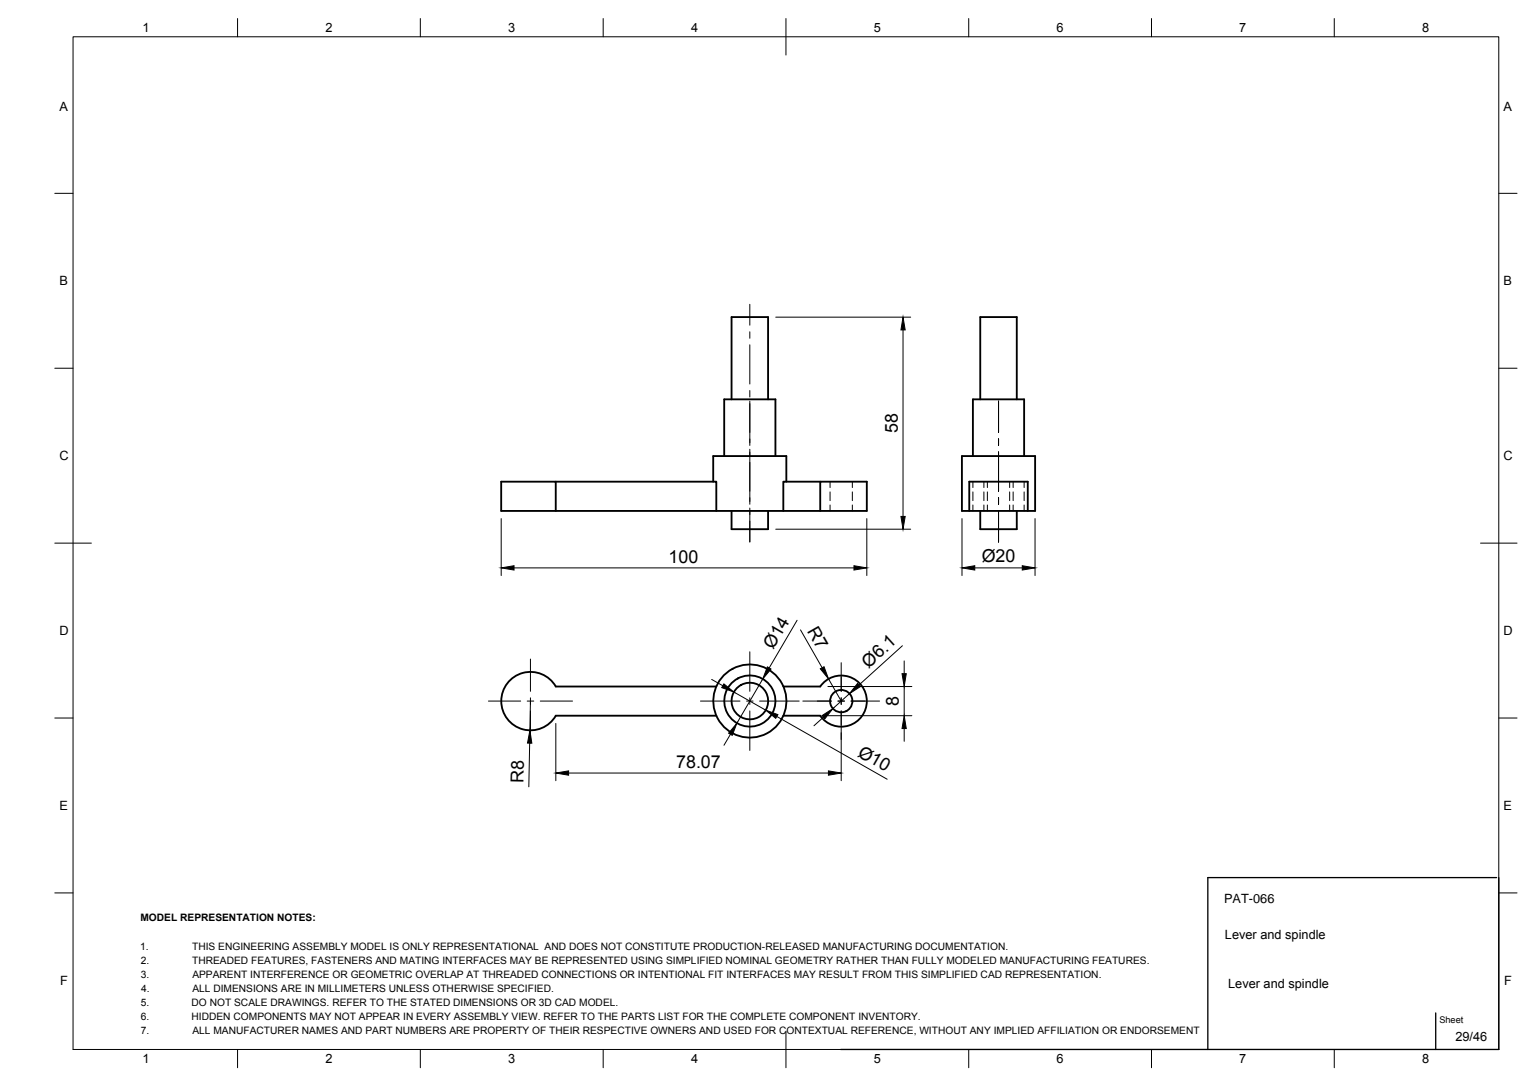
ISO-10303-21;
HEADER;
/* Generated by software containing ST-Developer
 * from STEP Tools, Inc. (www.steptools.com) 
 */

FILE_DESCRIPTION(
/* description */ ('Lever-operated bar clamp (toggle)'),
/* implementation_level */ '2;1');

FILE_NAME(
/* name */ 'Lever and spindle.step',
/* time_stamp */ '2026-10-28T03:25:02-07:00',
/* author */ (''),
/* organization */ (''),
/* preprocessor_version */ 'ST-DEVELOPER v20.2',
/* originating_system */ 'Autodesk Translation Framework v15.17.0.0',
/* authorisation */ '');

FILE_SCHEMA (('AUTOMOTIVE_DESIGN { 1 0 10303 214 3 1 1 }'));
ENDSEC;

DATA;
#10=MECHANICAL_DESIGN_GEOMETRIC_PRESENTATION_REPRESENTATION('',(#438),#12413);
#354=SHAPE_REPRESENTATION_RELATIONSHIP('SRR','None',#12596,#392);
#392=ADVANCED_BREP_SHAPE_REPRESENTATION('',(#483),#12393);
#438=STYLED_ITEM('',(#12862),#483);
#483=MANIFOLD_SOLID_BREP('Body1',#6599);
#610=FACE_BOUND('',#1653,.T.);
#611=FACE_BOUND('',#1654,.T.);
#612=FACE_BOUND('',#1661,.T.);
#613=FACE_BOUND('',#1664,.T.);
#614=FACE_BOUND('',#1667,.T.);
#785=PLANE('',#7551);
#786=PLANE('',#7557);
#787=PLANE('',#7558);
#788=PLANE('',#7560);
#789=PLANE('',#7563);
#790=PLANE('',#7564);
#791=PLANE('',#7566);
#792=PLANE('',#7567);
#793=PLANE('',#7571);
#794=PLANE('',#7579);
#795=PLANE('',#7580);
#1134=FACE_OUTER_BOUND('',#1650,.T.);
#1135=FACE_OUTER_BOUND('',#1651,.T.);
#1136=FACE_OUTER_BOUND('',#1652,.T.);
#1137=FACE_OUTER_BOUND('',#1655,.T.);
#1138=FACE_OUTER_BOUND('',#1656,.T.);
#1139=FACE_OUTER_BOUND('',#1657,.T.);
#1140=FACE_OUTER_BOUND('',#1658,.T.);
#1141=FACE_OUTER_BOUND('',#1659,.T.);
#1142=FACE_OUTER_BOUND('',#1660,.T.);
#1143=FACE_OUTER_BOUND('',#1662,.T.);
#1144=FACE_OUTER_BOUND('',#1663,.T.);
#1145=FACE_OUTER_BOUND('',#1665,.T.);
#1146=FACE_OUTER_BOUND('',#1666,.T.);
#1147=FACE_OUTER_BOUND('',#1668,.T.);
#1148=FACE_OUTER_BOUND('',#1669,.T.);
#1149=FACE_OUTER_BOUND('',#1670,.T.);
#1150=FACE_OUTER_BOUND('',#1671,.T.);
#1151=FACE_OUTER_BOUND('',#1672,.T.);
#1650=EDGE_LOOP('',(#5423,#5424,#5425,#5426));
#1651=EDGE_LOOP('',(#5427,#5428,#5429,#5430));
#1652=EDGE_LOOP('',(#5431,#5432,#5433,#5434,#5435,#5436,#5437,#5438,#5439));
#1653=EDGE_LOOP('',(#5440));
#1654=EDGE_LOOP('',(#5441));
#1655=EDGE_LOOP('',(#5442,#5443,#5444,#5445));
#1656=EDGE_LOOP('',(#5446,#5447,#5448,#5449));
#1657=EDGE_LOOP('',(#5450,#5451,#5452,#5453));
#1658=EDGE_LOOP('',(#5454,#5455,#5456,#5457));
#1659=EDGE_LOOP('',(#5458,#5459,#5460,#5461));
#1660=EDGE_LOOP('',(#5462,#5463,#5464,#5465));
#1661=EDGE_LOOP('',(#5466));
#1662=EDGE_LOOP('',(#5467,#5468,#5469,#5470));
#1663=EDGE_LOOP('',(#5471));
#1664=EDGE_LOOP('',(#5472));
#1665=EDGE_LOOP('',(#5473,#5474,#5475,#5476,#5477,#5478,#5479,#5480,#5481,
#5482,#5483,#5484));
#1666=EDGE_LOOP('',(#5485));
#1667=EDGE_LOOP('',(#5486));
#1668=EDGE_LOOP('',(#5487,#5488,#5489,#5490));
#1669=EDGE_LOOP('',(#5491,#5492,#5493,#5494));
#1670=EDGE_LOOP('',(#5495,#5496,#5497,#5498));
#1671=EDGE_LOOP('',(#5499));
#1672=EDGE_LOOP('',(#5500));
#2107=LINE('',#11508,#2548);
#2108=LINE('',#11513,#2549);
#2109=LINE('',#11517,#2550);
#2110=LINE('',#11521,#2551);
#2111=LINE('',#11527,#2552);
#2112=LINE('',#11531,#2553);
#2113=LINE('',#11534,#2554);
#2114=LINE('',#11539,#2555);
#2115=LINE('',#11540,#2556);
#2116=LINE('',#11543,#2557);
#2117=LINE('',#11546,#2558);
#2118=LINE('',#11549,#2559);
#2119=LINE('',#11552,#2560);
#2120=LINE('',#11555,#2561);
#2121=LINE('',#11556,#2562);
#2122=LINE('',#11559,#2563);
#2123=LINE('',#11562,#2564);
#2124=LINE('',#11569,#2565);
#2125=LINE('',#11576,#2566);
#2126=LINE('',#11579,#2567);
#2127=LINE('',#11584,#2568);
#2548=VECTOR('',#9166,0.305);
#2549=VECTOR('',#9171,1.);
#2550=VECTOR('',#9174,1.);
#2551=VECTOR('',#9179,1.);
#2552=VECTOR('',#9184,1.);
#2553=VECTOR('',#9187,1.);
#2554=VECTOR('',#9190,1.);
#2555=VECTOR('',#9195,1.);
#2556=VECTOR('',#9196,1.);
#2557=VECTOR('',#9199,1.);
#2558=VECTOR('',#9204,1.);
#2559=VECTOR('',#9207,1.);
#2560=VECTOR('',#9210,1.);
#2561=VECTOR('',#9213,1.);
#2562=VECTOR('',#9214,1.);
#2563=VECTOR('',#9217,1.);
#2564=VECTOR('',#9222,1.);
#2565=VECTOR('',#9231,1.);
#2566=VECTOR('',#9240,0.7);
#2567=VECTOR('',#9243,0.5);
#2568=VECTOR('',#9250,0.5);
#2960=CIRCLE('',#7546,0.305);
#2961=CIRCLE('',#7547,0.305);
#2962=CIRCLE('',#7549,0.8);
#2963=CIRCLE('',#7550,0.8);
#2964=CIRCLE('',#7552,1.);
#2965=CIRCLE('',#7553,1.);
#2966=CIRCLE('',#7554,0.7);
#2967=CIRCLE('',#7555,1.);
#2968=CIRCLE('',#7556,0.5);
#2969=CIRCLE('',#7559,1.);
#2970=CIRCLE('',#7562,0.7);
#2971=CIRCLE('',#7565,1.);
#2972=CIRCLE('',#7568,1.);
#2973=CIRCLE('',#7569,0.7);
#2974=CIRCLE('',#7572,0.7);
#2975=CIRCLE('',#7573,0.5);
#2976=CIRCLE('',#7576,0.5);
#2977=CIRCLE('',#7578,0.5);
#3415=VERTEX_POINT('',#11505);
#3416=VERTEX_POINT('',#11507);
#3417=VERTEX_POINT('',#11511);
#3418=VERTEX_POINT('',#11512);
#3419=VERTEX_POINT('',#11514);
#3420=VERTEX_POINT('',#11516);
#3421=VERTEX_POINT('',#11520);
#3422=VERTEX_POINT('',#11522);
#3423=VERTEX_POINT('',#11524);
#3424=VERTEX_POINT('',#11526);
#3425=VERTEX_POINT('',#11528);
#3426=VERTEX_POINT('',#11530);
#3427=VERTEX_POINT('',#11532);
#3428=VERTEX_POINT('',#11535);
#3429=VERTEX_POINT('',#11538);
#3430=VERTEX_POINT('',#11542);
#3431=VERTEX_POINT('',#11548);
#3432=VERTEX_POINT('',#11550);
#3433=VERTEX_POINT('',#11554);
#3434=VERTEX_POINT('',#11558);
#3435=VERTEX_POINT('',#11564);
#3436=VERTEX_POINT('',#11566);
#3437=VERTEX_POINT('',#11571);
#3438=VERTEX_POINT('',#11573);
#3439=VERTEX_POINT('',#11578);
#3440=VERTEX_POINT('',#11582);
#4116=EDGE_CURVE('',#3415,#3415,#2960,.T.);
#4117=EDGE_CURVE('',#3415,#3416,#2107,.T.);
#4118=EDGE_CURVE('',#3416,#3416,#2961,.T.);
#4119=EDGE_CURVE('',#3417,#3418,#2108,.T.);
#4120=EDGE_CURVE('',#3419,#3417,#2962,.T.);
#4121=EDGE_CURVE('',#3420,#3419,#2109,.T.);
#4122=EDGE_CURVE('',#3420,#3418,#2963,.T.);
#4123=EDGE_CURVE('',#3421,#3420,#2110,.T.);
#4124=EDGE_CURVE('',#3422,#3421,#2964,.T.);
#4125=EDGE_CURVE('',#3423,#3422,#2965,.T.);
#4126=EDGE_CURVE('',#3424,#3423,#2111,.T.);
#4127=EDGE_CURVE('',#3425,#3424,#2966,.T.);
#4128=EDGE_CURVE('',#3426,#3425,#2112,.T.);
#4129=EDGE_CURVE('',#3427,#3426,#2967,.T.);
#4130=EDGE_CURVE('',#3418,#3427,#2113,.T.);
#4131=EDGE_CURVE('',#3428,#3428,#2968,.T.);
#4132=EDGE_CURVE('',#3429,#3419,#2114,.T.);
#4133=EDGE_CURVE('',#3421,#3429,#2115,.T.);
#4134=EDGE_CURVE('',#3417,#3430,#2116,.T.);
#4135=EDGE_CURVE('',#3429,#3430,#2969,.T.);
#4136=EDGE_CURVE('',#3430,#3427,#2117,.T.);
#4137=EDGE_CURVE('',#3431,#3424,#2118,.T.);
#4138=EDGE_CURVE('',#3432,#3431,#2970,.T.);
#4139=EDGE_CURVE('',#3425,#3432,#2119,.T.);
#4140=EDGE_CURVE('',#3433,#3432,#2120,.T.);
#4141=EDGE_CURVE('',#3426,#3433,#2121,.T.);
#4142=EDGE_CURVE('',#3431,#3434,#2122,.T.);
#4143=EDGE_CURVE('',#3433,#3434,#2971,.T.);
#4144=EDGE_CURVE('',#3434,#3423,#2123,.T.);
#4145=EDGE_CURVE('',#3435,#3435,#2972,.T.);
#4146=EDGE_CURVE('',#3436,#3436,#2973,.T.);
#4147=EDGE_CURVE('',#3435,#3422,#2124,.T.);
#4148=EDGE_CURVE('',#3437,#3437,#2974,.T.);
#4149=EDGE_CURVE('',#3438,#3438,#2975,.T.);
#4150=EDGE_CURVE('',#3437,#3436,#2125,.T.);
#4151=EDGE_CURVE('',#3428,#3439,#2126,.T.);
#4152=EDGE_CURVE('',#3439,#3439,#2976,.T.);
#4153=EDGE_CURVE('',#3440,#3440,#2977,.T.);
#4154=EDGE_CURVE('',#3440,#3438,#2127,.T.);
#5423=ORIENTED_EDGE('',*,*,#4116,.F.);
#5424=ORIENTED_EDGE('',*,*,#4117,.T.);
#5425=ORIENTED_EDGE('',*,*,#4118,.F.);
#5426=ORIENTED_EDGE('',*,*,#4117,.F.);
#5427=ORIENTED_EDGE('',*,*,#4119,.F.);
#5428=ORIENTED_EDGE('',*,*,#4120,.F.);
#5429=ORIENTED_EDGE('',*,*,#4121,.F.);
#5430=ORIENTED_EDGE('',*,*,#4122,.T.);
#5431=ORIENTED_EDGE('',*,*,#4122,.F.);
#5432=ORIENTED_EDGE('',*,*,#4123,.F.);
#5433=ORIENTED_EDGE('',*,*,#4124,.F.);
#5434=ORIENTED_EDGE('',*,*,#4125,.F.);
#5435=ORIENTED_EDGE('',*,*,#4126,.F.);
#5436=ORIENTED_EDGE('',*,*,#4127,.F.);
#5437=ORIENTED_EDGE('',*,*,#4128,.F.);
#5438=ORIENTED_EDGE('',*,*,#4129,.F.);
#5439=ORIENTED_EDGE('',*,*,#4130,.F.);
#5440=ORIENTED_EDGE('',*,*,#4116,.T.);
#5441=ORIENTED_EDGE('',*,*,#4131,.F.);
#5442=ORIENTED_EDGE('',*,*,#4121,.T.);
#5443=ORIENTED_EDGE('',*,*,#4132,.F.);
#5444=ORIENTED_EDGE('',*,*,#4133,.F.);
#5445=ORIENTED_EDGE('',*,*,#4123,.T.);
#5446=ORIENTED_EDGE('',*,*,#4134,.T.);
#5447=ORIENTED_EDGE('',*,*,#4135,.F.);
#5448=ORIENTED_EDGE('',*,*,#4132,.T.);
#5449=ORIENTED_EDGE('',*,*,#4120,.T.);
#5450=ORIENTED_EDGE('',*,*,#4119,.T.);
#5451=ORIENTED_EDGE('',*,*,#4130,.T.);
#5452=ORIENTED_EDGE('',*,*,#4136,.F.);
#5453=ORIENTED_EDGE('',*,*,#4134,.F.);
#5454=ORIENTED_EDGE('',*,*,#4137,.F.);
#5455=ORIENTED_EDGE('',*,*,#4138,.F.);
#5456=ORIENTED_EDGE('',*,*,#4139,.F.);
#5457=ORIENTED_EDGE('',*,*,#4127,.T.);
#5458=ORIENTED_EDGE('',*,*,#4139,.T.);
#5459=ORIENTED_EDGE('',*,*,#4140,.F.);
#5460=ORIENTED_EDGE('',*,*,#4141,.F.);
#5461=ORIENTED_EDGE('',*,*,#4128,.T.);
#5462=ORIENTED_EDGE('',*,*,#4142,.T.);
#5463=ORIENTED_EDGE('',*,*,#4143,.F.);
#5464=ORIENTED_EDGE('',*,*,#4140,.T.);
#5465=ORIENTED_EDGE('',*,*,#4138,.T.);
#5466=ORIENTED_EDGE('',*,*,#4118,.T.);
#5467=ORIENTED_EDGE('',*,*,#4137,.T.);
#5468=ORIENTED_EDGE('',*,*,#4126,.T.);
#5469=ORIENTED_EDGE('',*,*,#4144,.F.);
#5470=ORIENTED_EDGE('',*,*,#4142,.F.);
#5471=ORIENTED_EDGE('',*,*,#4145,.T.);
#5472=ORIENTED_EDGE('',*,*,#4146,.F.);
#5473=ORIENTED_EDGE('',*,*,#4145,.F.);
#5474=ORIENTED_EDGE('',*,*,#4147,.T.);
#5475=ORIENTED_EDGE('',*,*,#4124,.T.);
#5476=ORIENTED_EDGE('',*,*,#4133,.T.);
#5477=ORIENTED_EDGE('',*,*,#4135,.T.);
#5478=ORIENTED_EDGE('',*,*,#4136,.T.);
#5479=ORIENTED_EDGE('',*,*,#4129,.T.);
#5480=ORIENTED_EDGE('',*,*,#4141,.T.);
#5481=ORIENTED_EDGE('',*,*,#4143,.T.);
#5482=ORIENTED_EDGE('',*,*,#4144,.T.);
#5483=ORIENTED_EDGE('',*,*,#4125,.T.);
#5484=ORIENTED_EDGE('',*,*,#4147,.F.);
#5485=ORIENTED_EDGE('',*,*,#4148,.T.);
#5486=ORIENTED_EDGE('',*,*,#4149,.F.);
#5487=ORIENTED_EDGE('',*,*,#4148,.F.);
#5488=ORIENTED_EDGE('',*,*,#4150,.T.);
#5489=ORIENTED_EDGE('',*,*,#4146,.T.);
#5490=ORIENTED_EDGE('',*,*,#4150,.F.);
#5491=ORIENTED_EDGE('',*,*,#4131,.T.);
#5492=ORIENTED_EDGE('',*,*,#4151,.T.);
#5493=ORIENTED_EDGE('',*,*,#4152,.T.);
#5494=ORIENTED_EDGE('',*,*,#4151,.F.);
#5495=ORIENTED_EDGE('',*,*,#4153,.F.);
#5496=ORIENTED_EDGE('',*,*,#4154,.T.);
#5497=ORIENTED_EDGE('',*,*,#4149,.T.);
#5498=ORIENTED_EDGE('',*,*,#4154,.F.);
#5499=ORIENTED_EDGE('',*,*,#4153,.T.);
#5500=ORIENTED_EDGE('',*,*,#4152,.F.);
#6116=CYLINDRICAL_SURFACE('',#7545,0.305);
#6117=CYLINDRICAL_SURFACE('',#7548,0.8);
#6118=CYLINDRICAL_SURFACE('',#7561,0.7);
#6119=CYLINDRICAL_SURFACE('',#7570,1.);
#6120=CYLINDRICAL_SURFACE('',#7574,0.7);
#6121=CYLINDRICAL_SURFACE('',#7575,0.5);
#6122=CYLINDRICAL_SURFACE('',#7577,0.5);
#6409=ADVANCED_FACE('',(#1134),#6116,.F.);
#6410=ADVANCED_FACE('',(#1135),#6117,.T.);
#6411=ADVANCED_FACE('',(#1136,#610,#611),#785,.F.);
#6412=ADVANCED_FACE('',(#1137),#786,.T.);
#6413=ADVANCED_FACE('',(#1138),#787,.T.);
#6414=ADVANCED_FACE('',(#1139),#788,.T.);
#6415=ADVANCED_FACE('',(#1140),#6118,.T.);
#6416=ADVANCED_FACE('',(#1141),#789,.T.);
#6417=ADVANCED_FACE('',(#1142,#612),#790,.T.);
#6418=ADVANCED_FACE('',(#1143),#791,.T.);
#6419=ADVANCED_FACE('',(#1144,#613),#792,.T.);
#6420=ADVANCED_FACE('',(#1145),#6119,.T.);
#6421=ADVANCED_FACE('',(#1146,#614),#793,.T.);
#6422=ADVANCED_FACE('',(#1147),#6120,.T.);
#6423=ADVANCED_FACE('',(#1148),#6121,.T.);
#6424=ADVANCED_FACE('',(#1149),#6122,.T.);
#6425=ADVANCED_FACE('',(#1150),#794,.T.);
#6426=ADVANCED_FACE('',(#1151),#795,.F.);
#6599=CLOSED_SHELL('',(#6409,#6410,#6411,#6412,#6413,#6414,#6415,#6416,
#6417,#6418,#6419,#6420,#6421,#6422,#6423,#6424,#6425,#6426));
#7544=AXIS2_PLACEMENT_3D('',#11503,#9160,#9161);
#7545=AXIS2_PLACEMENT_3D('',#11504,#9162,#9163);
#7546=AXIS2_PLACEMENT_3D('',#11506,#9164,#9165);
#7547=AXIS2_PLACEMENT_3D('',#11509,#9167,#9168);
#7548=AXIS2_PLACEMENT_3D('',#11510,#9169,#9170);
#7549=AXIS2_PLACEMENT_3D('',#11515,#9172,#9173);
#7550=AXIS2_PLACEMENT_3D('',#11518,#9175,#9176);
#7551=AXIS2_PLACEMENT_3D('',#11519,#9177,#9178);
#7552=AXIS2_PLACEMENT_3D('',#11523,#9180,#9181);
#7553=AXIS2_PLACEMENT_3D('',#11525,#9182,#9183);
#7554=AXIS2_PLACEMENT_3D('',#11529,#9185,#9186);
#7555=AXIS2_PLACEMENT_3D('',#11533,#9188,#9189);
#7556=AXIS2_PLACEMENT_3D('',#11536,#9191,#9192);
#7557=AXIS2_PLACEMENT_3D('',#11537,#9193,#9194);
#7558=AXIS2_PLACEMENT_3D('',#11541,#9197,#9198);
#7559=AXIS2_PLACEMENT_3D('',#11544,#9200,#9201);
#7560=AXIS2_PLACEMENT_3D('',#11545,#9202,#9203);
#7561=AXIS2_PLACEMENT_3D('',#11547,#9205,#9206);
#7562=AXIS2_PLACEMENT_3D('',#11551,#9208,#9209);
#7563=AXIS2_PLACEMENT_3D('',#11553,#9211,#9212);
#7564=AXIS2_PLACEMENT_3D('',#11557,#9215,#9216);
#7565=AXIS2_PLACEMENT_3D('',#11560,#9218,#9219);
#7566=AXIS2_PLACEMENT_3D('',#11561,#9220,#9221);
#7567=AXIS2_PLACEMENT_3D('',#11563,#9223,#9224);
#7568=AXIS2_PLACEMENT_3D('',#11565,#9225,#9226);
#7569=AXIS2_PLACEMENT_3D('',#11567,#9227,#9228);
#7570=AXIS2_PLACEMENT_3D('',#11568,#9229,#9230);
#7571=AXIS2_PLACEMENT_3D('',#11570,#9232,#9233);
#7572=AXIS2_PLACEMENT_3D('',#11572,#9234,#9235);
#7573=AXIS2_PLACEMENT_3D('',#11574,#9236,#9237);
#7574=AXIS2_PLACEMENT_3D('',#11575,#9238,#9239);
#7575=AXIS2_PLACEMENT_3D('',#11577,#9241,#9242);
#7576=AXIS2_PLACEMENT_3D('',#11580,#9244,#9245);
#7577=AXIS2_PLACEMENT_3D('',#11581,#9246,#9247);
#7578=AXIS2_PLACEMENT_3D('',#11583,#9248,#9249);
#7579=AXIS2_PLACEMENT_3D('',#11585,#9251,#9252);
#7580=AXIS2_PLACEMENT_3D('',#11586,#9253,#9254);
#9160=DIRECTION('axis',(0.,0.,1.));
#9161=DIRECTION('refdir',(1.,0.,0.));
#9162=DIRECTION('center_axis',(0.,1.,0.));
#9163=DIRECTION('ref_axis',(1.,0.,0.));
#9164=DIRECTION('center_axis',(0.,1.,0.));
#9165=DIRECTION('ref_axis',(1.,0.,0.));
#9166=DIRECTION('',(0.,1.,0.));
#9167=DIRECTION('center_axis',(0.,-1.,0.));
#9168=DIRECTION('ref_axis',(1.,0.,0.));
#9169=DIRECTION('center_axis',(0.,1.,0.));
#9170=DIRECTION('ref_axis',(-0.46947156278589,0.,0.882947592858928));
#9171=DIRECTION('',(0.,-1.,0.));
#9172=DIRECTION('center_axis',(0.,1.,0.));
#9173=DIRECTION('ref_axis',(1.,0.,0.));
#9174=DIRECTION('',(0.,1.,0.));
#9175=DIRECTION('center_axis',(0.,1.,0.));
#9176=DIRECTION('ref_axis',(1.,0.,0.));
#9177=DIRECTION('center_axis',(0.,1.,0.));
#9178=DIRECTION('ref_axis',(1.,0.,0.));
#9179=DIRECTION('',(-0.469471562785891,0.,0.882947592858927));
#9180=DIRECTION('center_axis',(0.,1.,0.));
#9181=DIRECTION('ref_axis',(1.,0.,0.));
#9182=DIRECTION('center_axis',(0.,1.,0.));
#9183=DIRECTION('ref_axis',(1.,0.,0.));
#9184=DIRECTION('',(-0.469471562785891,0.,0.882947592858927));
#9185=DIRECTION('center_axis',(0.,1.,0.));
#9186=DIRECTION('ref_axis',(1.,0.,0.));
#9187=DIRECTION('',(0.469471562785891,0.,-0.882947592858927));
#9188=DIRECTION('center_axis',(0.,1.,0.));
#9189=DIRECTION('ref_axis',(1.,0.,0.));
#9190=DIRECTION('',(0.469471562785891,0.,-0.882947592858927));
#9191=DIRECTION('center_axis',(0.,-1.,0.));
#9192=DIRECTION('ref_axis',(1.,0.,0.));
#9193=DIRECTION('center_axis',(-0.882947592858927,0.,-0.469471562785891));
#9194=DIRECTION('ref_axis',(-0.469471562785891,0.,0.882947592858927));
#9195=DIRECTION('',(-0.469471562785891,0.,0.882947592858927));
#9196=DIRECTION('',(0.,1.,0.));
#9197=DIRECTION('center_axis',(0.,1.,0.));
#9198=DIRECTION('ref_axis',(0.,0.,1.));
#9199=DIRECTION('',(0.469471562785891,0.,-0.882947592858927));
#9200=DIRECTION('center_axis',(0.,1.,0.));
#9201=DIRECTION('ref_axis',(1.,0.,0.));
#9202=DIRECTION('center_axis',(0.882947592858927,0.,0.469471562785891));
#9203=DIRECTION('ref_axis',(0.469471562785891,0.,-0.882947592858927));
#9204=DIRECTION('',(0.,-1.,0.));
#9205=DIRECTION('center_axis',(0.,1.,0.));
#9206=DIRECTION('ref_axis',(0.46947156278589,0.,-0.882947592858927));
#9207=DIRECTION('',(0.,-1.,0.));
#9208=DIRECTION('center_axis',(0.,1.,0.));
#9209=DIRECTION('ref_axis',(1.,0.,0.));
#9210=DIRECTION('',(0.,1.,0.));
#9211=DIRECTION('center_axis',(0.882947592858927,0.,0.469471562785891));
#9212=DIRECTION('ref_axis',(0.469471562785891,0.,-0.882947592858927));
#9213=DIRECTION('',(0.469471562785891,0.,-0.882947592858927));
#9214=DIRECTION('',(0.,1.,0.));
#9215=DIRECTION('center_axis',(0.,1.,0.));
#9216=DIRECTION('ref_axis',(0.,0.,1.));
#9217=DIRECTION('',(-0.469471562785891,0.,0.882947592858927));
#9218=DIRECTION('center_axis',(0.,1.,0.));
#9219=DIRECTION('ref_axis',(1.,0.,0.));
#9220=DIRECTION('center_axis',(-0.882947592858927,0.,-0.469471562785891));
#9221=DIRECTION('ref_axis',(-0.469471562785891,0.,0.882947592858927));
#9222=DIRECTION('',(0.,-1.,0.));
#9223=DIRECTION('center_axis',(0.,1.,0.));
#9224=DIRECTION('ref_axis',(1.,0.,0.));
#9225=DIRECTION('center_axis',(0.,1.,0.));
#9226=DIRECTION('ref_axis',(1.,0.,0.));
#9227=DIRECTION('center_axis',(0.,1.,0.));
#9228=DIRECTION('ref_axis',(1.,0.,0.));
#9229=DIRECTION('center_axis',(0.,1.,0.));
#9230=DIRECTION('ref_axis',(1.,0.,0.));
#9231=DIRECTION('',(0.,-1.,0.));
#9232=DIRECTION('center_axis',(0.,1.,0.));
#9233=DIRECTION('ref_axis',(1.,0.,0.));
#9234=DIRECTION('center_axis',(0.,1.,0.));
#9235=DIRECTION('ref_axis',(1.,0.,0.));
#9236=DIRECTION('center_axis',(0.,1.,0.));
#9237=DIRECTION('ref_axis',(1.,0.,0.));
#9238=DIRECTION('center_axis',(0.,1.,0.));
#9239=DIRECTION('ref_axis',(1.,0.,0.));
#9240=DIRECTION('',(0.,-1.,0.));
#9241=DIRECTION('center_axis',(0.,1.,0.));
#9242=DIRECTION('ref_axis',(1.,0.,0.));
#9243=DIRECTION('',(0.,-1.,0.));
#9244=DIRECTION('center_axis',(0.,1.,0.));
#9245=DIRECTION('ref_axis',(1.,0.,0.));
#9246=DIRECTION('center_axis',(0.,1.,0.));
#9247=DIRECTION('ref_axis',(1.,0.,0.));
#9248=DIRECTION('center_axis',(0.,1.,0.));
#9249=DIRECTION('ref_axis',(1.,0.,0.));
#9250=DIRECTION('',(0.,-1.,0.));
#9251=DIRECTION('center_axis',(0.,1.,0.));
#9252=DIRECTION('ref_axis',(1.,0.,0.));
#9253=DIRECTION('center_axis',(0.,1.,0.));
#9254=DIRECTION('ref_axis',(1.,0.,0.));
#11503=CARTESIAN_POINT('',(0.,0.,0.));
#11504=CARTESIAN_POINT('Origin',(-2.82632109303527,-3.6,8.79263101785268));
#11505=CARTESIAN_POINT('',(-3.13132109303527,-3.5,8.79263101785268));
#11506=CARTESIAN_POINT('Origin',(-2.82632109303527,-3.5,8.79263101785268));
#11507=CARTESIAN_POINT('',(-3.13132109303527,-2.7,8.79263101785268));
#11508=CARTESIAN_POINT('',(-3.13132109303527,-3.6,8.79263101785268));
#11509=CARTESIAN_POINT('Origin',(-2.82632109303527,-2.7,8.79263101785268));
#11510=CARTESIAN_POINT('Origin',(-6.81682937671534,-3.5,16.2976855571536));
#11511=CARTESIAN_POINT('',(-6.1383908997902,-2.7,15.873750145767));
#11512=CARTESIAN_POINT('',(-6.1383908997902,-3.5,15.873750145767));
#11513=CARTESIAN_POINT('',(-6.1383908997902,-3.5,15.873750145767));
#11514=CARTESIAN_POINT('',(-6.84474897407734,-2.7,15.4981728955383));
#11515=CARTESIAN_POINT('Origin',(-6.81682937671534,-2.7,16.2976855571536));
#11516=CARTESIAN_POINT('',(-6.84474897407734,-3.5,15.4981728955383));
#11517=CARTESIAN_POINT('',(-6.84474897407734,-3.5,15.4981728955383));
#11518=CARTESIAN_POINT('Origin',(-6.81682937671534,-3.5,16.2976855571536));
#11519=CARTESIAN_POINT('Origin',(-4.,-3.5,11.));
#11520=CARTESIAN_POINT('',(-4.78345683176268,-3.5,11.6214462106767));
#11521=CARTESIAN_POINT('',(-4.35317903714357,-3.5,10.8122113748856));
#11522=CARTESIAN_POINT('',(-5.,-3.5,11.));
#11523=CARTESIAN_POINT('Origin',(-4.,-3.5,11.));
#11524=CARTESIAN_POINT('',(-3.92290124252446,-3.5,10.0029765390946));
#11525=CARTESIAN_POINT('Origin',(-4.,-3.5,11.));
#11526=CARTESIAN_POINT('',(-3.44919101049801,-3.5,9.11205716881713));
#11527=CARTESIAN_POINT('',(-3.17950013017884,-3.5,8.60484239273833));
#11528=CARTESIAN_POINT('',(-2.74283293621087,-3.5,9.48763441904585));
#11529=CARTESIAN_POINT('Origin',(-2.82632109303527,-3.5,8.79263101785268));
#11530=CARTESIAN_POINT('',(-3.21654316823732,-3.5,10.3785537893233));
#11531=CARTESIAN_POINT('',(-3.64682096285643,-3.5,11.1877886251144));
#11532=CARTESIAN_POINT('',(-4.07709875747554,-3.5,11.9970234609054));
#11533=CARTESIAN_POINT('Origin',(-4.,-3.5,11.));
#11534=CARTESIAN_POINT('',(-6.46365033957177,-3.5,16.4854741822679));
#11535=CARTESIAN_POINT('',(-4.5,-3.5,11.));
#11536=CARTESIAN_POINT('Origin',(-4.,-3.5,11.));
#11537=CARTESIAN_POINT('Origin',(-4.35317903714357,-3.5,10.8122113748856));
#11538=CARTESIAN_POINT('',(-4.78345683176268,-2.7,11.6214462106767));
#11539=CARTESIAN_POINT('',(-4.35317903714357,-2.7,10.8122113748856));
#11540=CARTESIAN_POINT('',(-4.78345683176268,-3.5,11.6214462106767));
#11541=CARTESIAN_POINT('Origin',(-5.40841468835767,-2.7,13.6488427785768));
#11542=CARTESIAN_POINT('',(-4.07709875747554,-2.7,11.9970234609054));
#11543=CARTESIAN_POINT('',(-6.46365033957177,-2.7,16.4854741822679));
#11544=CARTESIAN_POINT('Origin',(-4.,-2.7,11.));
#11545=CARTESIAN_POINT('Origin',(-6.46365033957177,-3.5,16.4854741822679));
#11546=CARTESIAN_POINT('',(-4.07709875747554,-3.5,11.9970234609054));
#11547=CARTESIAN_POINT('Origin',(-2.82632109303527,-3.5,8.79263101785268));
#11548=CARTESIAN_POINT('',(-3.44919101049801,-2.7,9.11205716881713));
#11549=CARTESIAN_POINT('',(-3.44919101049801,-3.5,9.11205716881713));
#11550=CARTESIAN_POINT('',(-2.74283293621087,-2.7,9.48763441904585));
#11551=CARTESIAN_POINT('Origin',(-2.82632109303527,-2.7,8.79263101785268));
#11552=CARTESIAN_POINT('',(-2.74283293621087,-3.5,9.48763441904585));
#11553=CARTESIAN_POINT('Origin',(-3.64682096285643,-3.5,11.1877886251144));
#11554=CARTESIAN_POINT('',(-3.21654316823732,-2.7,10.3785537893233));
#11555=CARTESIAN_POINT('',(-3.64682096285643,-2.7,11.1877886251144));
#11556=CARTESIAN_POINT('',(-3.21654316823732,-3.5,10.3785537893233));
#11557=CARTESIAN_POINT('Origin',(-3.41316054651764,-2.7,9.89631550892634));
#11558=CARTESIAN_POINT('',(-3.92290124252446,-2.7,10.0029765390946));
#11559=CARTESIAN_POINT('',(-3.17950013017884,-2.7,8.60484239273833));
#11560=CARTESIAN_POINT('Origin',(-4.,-2.7,11.));
#11561=CARTESIAN_POINT('Origin',(-3.17950013017884,-3.5,8.60484239273833));
#11562=CARTESIAN_POINT('',(-3.92290124252446,-3.5,10.0029765390946));
#11563=CARTESIAN_POINT('Origin',(-4.,-2.,11.));
#11564=CARTESIAN_POINT('',(-5.,-2.,11.));
#11565=CARTESIAN_POINT('Origin',(-4.,-2.,11.));
#11566=CARTESIAN_POINT('',(-4.7,-2.,11.));
#11567=CARTESIAN_POINT('Origin',(-4.,-2.,11.));
#11568=CARTESIAN_POINT('Origin',(-4.,-3.5,11.));
#11569=CARTESIAN_POINT('',(-5.,-3.5,11.));
#11570=CARTESIAN_POINT('Origin',(-4.,-0.45,11.));
#11571=CARTESIAN_POINT('',(-4.7,-0.45,11.));
#11572=CARTESIAN_POINT('Origin',(-4.,-0.45,11.));
#11573=CARTESIAN_POINT('',(-4.5,-0.45,11.));
#11574=CARTESIAN_POINT('Origin',(-4.,-0.45,11.));
#11575=CARTESIAN_POINT('Origin',(-4.,-2.,11.));
#11576=CARTESIAN_POINT('',(-4.7,-2.,11.));
#11577=CARTESIAN_POINT('Origin',(-4.,-4.,11.));
#11578=CARTESIAN_POINT('',(-4.5,-4.,11.));
#11579=CARTESIAN_POINT('',(-4.5,-4.,11.));
#11580=CARTESIAN_POINT('Origin',(-4.,-4.,11.));
#11581=CARTESIAN_POINT('Origin',(-4.,-4.,11.));
#11582=CARTESIAN_POINT('',(-4.5,1.8,11.));
#11583=CARTESIAN_POINT('Origin',(-4.,1.8,11.));
#11584=CARTESIAN_POINT('',(-4.5,-4.,11.));
#11585=CARTESIAN_POINT('Origin',(-4.,1.8,11.));
#11586=CARTESIAN_POINT('Origin',(-4.,-4.,11.));
#12347=UNCERTAINTY_MEASURE_WITH_UNIT(LENGTH_MEASURE(0.001),#12414,
'DISTANCE_ACCURACY_VALUE',
'Maximum model space distance between geometric entities at asserted c
onnectivities');
#12367=UNCERTAINTY_MEASURE_WITH_UNIT(LENGTH_MEASURE(0.001),#12414,
'DISTANCE_ACCURACY_VALUE',
'Maximum model space distance between geometric entities at asserted c
onnectivities');
#12393=(
GEOMETRIC_REPRESENTATION_CONTEXT(3)
GLOBAL_UNCERTAINTY_ASSIGNED_CONTEXT((#12347))
GLOBAL_UNIT_ASSIGNED_CONTEXT((#12414,#12416,#12417))
REPRESENTATION_CONTEXT('','3D')
);
#12413=(
GEOMETRIC_REPRESENTATION_CONTEXT(3)
GLOBAL_UNCERTAINTY_ASSIGNED_CONTEXT((#12367))
GLOBAL_UNIT_ASSIGNED_CONTEXT((#12414,#12416,#12417))
REPRESENTATION_CONTEXT('','3D')
);
#12414=(
LENGTH_UNIT()
NAMED_UNIT(*)
SI_UNIT(.CENTI.,.METRE.)
);
#12416=(
NAMED_UNIT(*)
PLANE_ANGLE_UNIT()
SI_UNIT($,.RADIAN.)
);
#12417=(
NAMED_UNIT(*)
SI_UNIT($,.STERADIAN.)
SOLID_ANGLE_UNIT()
);
#12443=SHAPE_DEFINITION_REPRESENTATION(#12495,#12596);
#12495=PRODUCT_DEFINITION_SHAPE('',$,#12642);
#12596=SHAPE_REPRESENTATION('',(#7544),#12393);
#12616=PRODUCT_DEFINITION_CONTEXT('part definition',#12753,'design');
#12642=PRODUCT_DEFINITION('Lever and spindle','Lever and spindle',#12687,
#12616);
#12687=PRODUCT_DEFINITION_FORMATION('',$,#12780);
#12753=APPLICATION_CONTEXT(
'Core Data for Automotive Mechanical Design Process');
#12754=PRODUCT_CONTEXT('part definition',#12753,'mechanical');
#12780=PRODUCT('Lever and spindle','Lever and spindle',
'Lever and spindle',(#12754));
#12856=COLOUR_RGB('Sky Blue',0.24,0.69,0.87);
#12857=FILL_AREA_STYLE_COLOUR('',#12856);
#12858=FILL_AREA_STYLE('',(#12857));
#12859=SURFACE_STYLE_FILL_AREA(#12858);
#12860=SURFACE_SIDE_STYLE('',(#12859));
#12861=SURFACE_STYLE_USAGE(.BOTH.,#12860);
#12862=PRESENTATION_STYLE_ASSIGNMENT((#12861));
ENDSEC;
END-ISO-10303-21;
